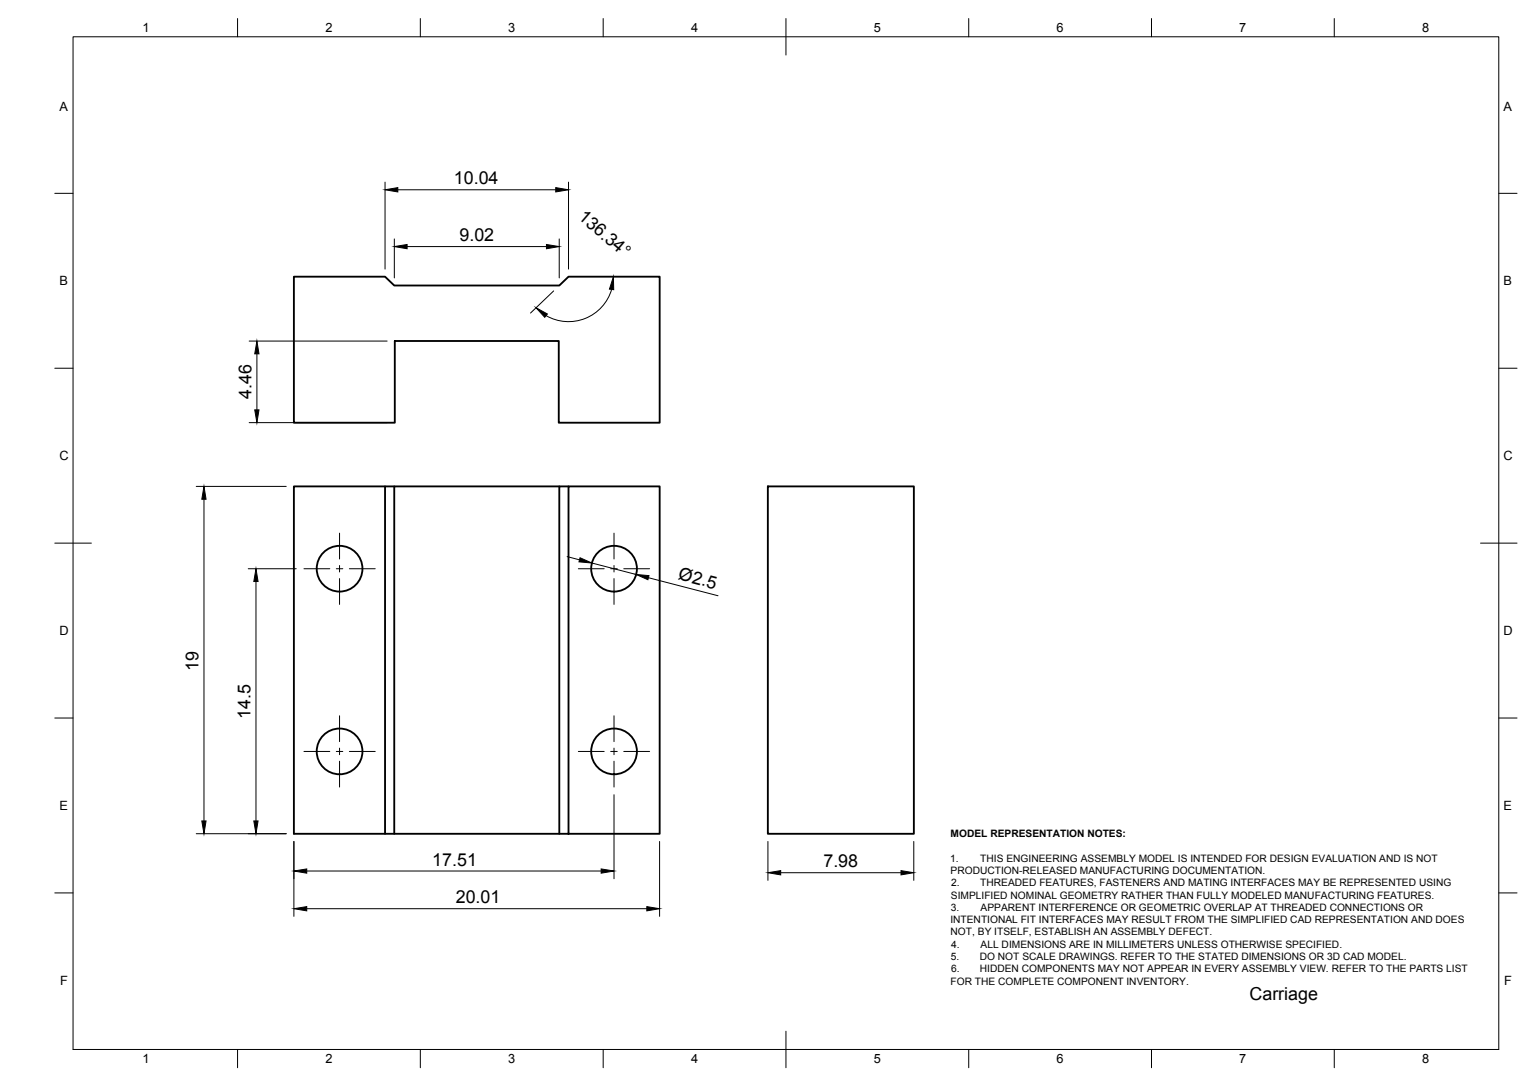
ISO-10303-21;
HEADER;
/* Generated by software containing ST-Developer
 * from STEP Tools, Inc. (www.steptools.com) 
 */

FILE_DESCRIPTION(
/* description */ (''),
/* implementation_level */ '2;1');

FILE_NAME(
/* name */ 'Carriage.step',
/* time_stamp */ '2026-10-06T13:23:02-07:00',
/* author */ (''),
/* organization */ (''),
/* preprocessor_version */ 'ST-DEVELOPER v20.2',
/* originating_system */ 'Autodesk Translation Framework v15.15.0.0',
/* authorisation */ '');

FILE_SCHEMA (('AUTOMOTIVE_DESIGN { 1 0 10303 214 3 1 1 }'));
ENDSEC;

DATA;
#10=MECHANICAL_DESIGN_GEOMETRIC_PRESENTATION_REPRESENTATION('',(#76),#4994);
#56=SHAPE_REPRESENTATION_RELATIONSHIP('SRR','None',#5037,#66);
#66=ADVANCED_BREP_SHAPE_REPRESENTATION('',(#86),#4989);
#76=STYLED_ITEM('',(#5092),#86);
#86=MANIFOLD_SOLID_BREP('Body1',#2916);
#111=CYLINDRICAL_SURFACE('',#3204,1.25);
#112=CYLINDRICAL_SURFACE('',#3208,1.25);
#113=CYLINDRICAL_SURFACE('',#3212,1.25);
#114=CYLINDRICAL_SURFACE('',#3216,1.25);
#146=FACE_BOUND('',#625,.T.);
#147=FACE_BOUND('',#626,.T.);
#148=FACE_BOUND('',#631,.T.);
#149=FACE_BOUND('',#632,.T.);
#241=PLANE('',#3207);
#242=PLANE('',#3211);
#243=PLANE('',#3215);
#244=PLANE('',#3219);
#245=PLANE('',#3220);
#246=PLANE('',#3221);
#247=PLANE('',#3222);
#248=PLANE('',#3223);
#249=PLANE('',#3224);
#250=PLANE('',#3225);
#251=PLANE('',#3226);
#252=PLANE('',#3227);
#253=PLANE('',#3228);
#254=PLANE('',#3229);
#255=PLANE('',#3230);
#256=PLANE('',#3231);
#257=PLANE('',#3232);
#258=PLANE('',#3233);
#411=FACE_OUTER_BOUND('',#612,.T.);
#412=FACE_OUTER_BOUND('',#613,.T.);
#413=FACE_OUTER_BOUND('',#614,.T.);
#414=FACE_OUTER_BOUND('',#615,.T.);
#415=FACE_OUTER_BOUND('',#616,.T.);
#416=FACE_OUTER_BOUND('',#617,.T.);
#417=FACE_OUTER_BOUND('',#618,.T.);
#418=FACE_OUTER_BOUND('',#619,.T.);
#419=FACE_OUTER_BOUND('',#620,.T.);
#420=FACE_OUTER_BOUND('',#621,.T.);
#421=FACE_OUTER_BOUND('',#622,.T.);
#422=FACE_OUTER_BOUND('',#623,.T.);
#423=FACE_OUTER_BOUND('',#624,.T.);
#424=FACE_OUTER_BOUND('',#627,.T.);
#425=FACE_OUTER_BOUND('',#628,.T.);
#426=FACE_OUTER_BOUND('',#629,.T.);
#427=FACE_OUTER_BOUND('',#630,.T.);
#428=FACE_OUTER_BOUND('',#633,.T.);
#429=FACE_OUTER_BOUND('',#634,.T.);
#430=FACE_OUTER_BOUND('',#635,.T.);
#431=FACE_OUTER_BOUND('',#636,.T.);
#432=FACE_OUTER_BOUND('',#637,.T.);
#612=EDGE_LOOP('',(#2388,#2389,#2390,#2391));
#613=EDGE_LOOP('',(#2392));
#614=EDGE_LOOP('',(#2393,#2394,#2395,#2396));
#615=EDGE_LOOP('',(#2397));
#616=EDGE_LOOP('',(#2398,#2399,#2400,#2401));
#617=EDGE_LOOP('',(#2402));
#618=EDGE_LOOP('',(#2403,#2404,#2405,#2406));
#619=EDGE_LOOP('',(#2407));
#620=EDGE_LOOP('',(#2408,#2409,#2410,#2411,#2412,#2413,#2414,#2415,#2416,
#2417,#2418,#2419));
#621=EDGE_LOOP('',(#2420,#2421,#2422,#2423));
#622=EDGE_LOOP('',(#2424,#2425,#2426,#2427));
#623=EDGE_LOOP('',(#2428,#2429,#2430,#2431));
#624=EDGE_LOOP('',(#2432,#2433,#2434,#2435));
#625=EDGE_LOOP('',(#2436));
#626=EDGE_LOOP('',(#2437));
#627=EDGE_LOOP('',(#2438,#2439,#2440,#2441));
#628=EDGE_LOOP('',(#2442,#2443,#2444,#2445));
#629=EDGE_LOOP('',(#2446,#2447,#2448,#2449));
#630=EDGE_LOOP('',(#2450,#2451,#2452,#2453));
#631=EDGE_LOOP('',(#2454));
#632=EDGE_LOOP('',(#2455));
#633=EDGE_LOOP('',(#2456,#2457,#2458,#2459));
#634=EDGE_LOOP('',(#2460,#2461,#2462,#2463));
#635=EDGE_LOOP('',(#2464,#2465,#2466,#2467));
#636=EDGE_LOOP('',(#2468,#2469,#2470,#2471));
#637=EDGE_LOOP('',(#2472,#2473,#2474,#2475,#2476,#2477,#2478,#2479,#2480,
#2481,#2482,#2483));
#851=LINE('',#4611,#1144);
#852=LINE('',#4618,#1145);
#853=LINE('',#4625,#1146);
#854=LINE('',#4632,#1147);
#855=LINE('',#4638,#1148);
#856=LINE('',#4640,#1149);
#857=LINE('',#4642,#1150);
#858=LINE('',#4644,#1151);
#859=LINE('',#4646,#1152);
#860=LINE('',#4648,#1153);
#861=LINE('',#4650,#1154);
#862=LINE('',#4652,#1155);
#863=LINE('',#4654,#1156);
#864=LINE('',#4656,#1157);
#865=LINE('',#4658,#1158);
#866=LINE('',#4659,#1159);
#867=LINE('',#4662,#1160);
#868=LINE('',#4664,#1161);
#869=LINE('',#4665,#1162);
#870=LINE('',#4668,#1163);
#871=LINE('',#4669,#1164);
#872=LINE('',#4672,#1165);
#873=LINE('',#4673,#1166);
#874=LINE('',#4676,#1167);
#875=LINE('',#4677,#1168);
#876=LINE('',#4680,#1169);
#877=LINE('',#4681,#1170);
#878=LINE('',#4684,#1171);
#879=LINE('',#4685,#1172);
#880=LINE('',#4688,#1173);
#881=LINE('',#4689,#1174);
#882=LINE('',#4692,#1175);
#883=LINE('',#4693,#1176);
#884=LINE('',#4696,#1177);
#885=LINE('',#4697,#1178);
#886=LINE('',#4700,#1179);
#887=LINE('',#4701,#1180);
#888=LINE('',#4704,#1181);
#889=LINE('',#4705,#1182);
#890=LINE('',#4707,#1183);
#1144=VECTOR('',#3809,1.25);
#1145=VECTOR('',#3818,1.25);
#1146=VECTOR('',#3827,1.25);
#1147=VECTOR('',#3836,1.25);
#1148=VECTOR('',#3843,10.);
#1149=VECTOR('',#3844,10.);
#1150=VECTOR('',#3845,10.);
#1151=VECTOR('',#3846,10.);
#1152=VECTOR('',#3847,10.);
#1153=VECTOR('',#3848,10.);
#1154=VECTOR('',#3849,10.);
#1155=VECTOR('',#3850,10.);
#1156=VECTOR('',#3851,10.);
#1157=VECTOR('',#3852,10.);
#1158=VECTOR('',#3853,10.);
#1159=VECTOR('',#3854,10.);
#1160=VECTOR('',#3857,10.);
#1161=VECTOR('',#3858,10.);
#1162=VECTOR('',#3859,10.);
#1163=VECTOR('',#3862,10.);
#1164=VECTOR('',#3863,10.);
#1165=VECTOR('',#3866,10.);
#1166=VECTOR('',#3867,10.);
#1167=VECTOR('',#3870,10.);
#1168=VECTOR('',#3871,10.);
#1169=VECTOR('',#3874,10.);
#1170=VECTOR('',#3875,10.);
#1171=VECTOR('',#3878,10.);
#1172=VECTOR('',#3879,10.);
#1173=VECTOR('',#3882,10.);
#1174=VECTOR('',#3883,10.);
#1175=VECTOR('',#3886,10.);
#1176=VECTOR('',#3887,10.);
#1177=VECTOR('',#3890,10.);
#1178=VECTOR('',#3891,10.);
#1179=VECTOR('',#3894,10.);
#1180=VECTOR('',#3895,10.);
#1181=VECTOR('',#3898,10.);
#1182=VECTOR('',#3899,10.);
#1183=VECTOR('',#3902,10.);
#1345=CIRCLE('',#3205,1.25);
#1346=CIRCLE('',#3206,1.25);
#1347=CIRCLE('',#3209,1.25);
#1348=CIRCLE('',#3210,1.25);
#1349=CIRCLE('',#3213,1.25);
#1350=CIRCLE('',#3214,1.25);
#1351=CIRCLE('',#3217,1.25);
#1352=CIRCLE('',#3218,1.25);
#1490=VERTEX_POINT('',#4608);
#1491=VERTEX_POINT('',#4610);
#1492=VERTEX_POINT('',#4615);
#1493=VERTEX_POINT('',#4617);
#1494=VERTEX_POINT('',#4622);
#1495=VERTEX_POINT('',#4624);
#1496=VERTEX_POINT('',#4629);
#1497=VERTEX_POINT('',#4631);
#1498=VERTEX_POINT('',#4636);
#1499=VERTEX_POINT('',#4637);
#1500=VERTEX_POINT('',#4639);
#1501=VERTEX_POINT('',#4641);
#1502=VERTEX_POINT('',#4643);
#1503=VERTEX_POINT('',#4645);
#1504=VERTEX_POINT('',#4647);
#1505=VERTEX_POINT('',#4649);
#1506=VERTEX_POINT('',#4651);
#1507=VERTEX_POINT('',#4653);
#1508=VERTEX_POINT('',#4655);
#1509=VERTEX_POINT('',#4657);
#1510=VERTEX_POINT('',#4661);
#1511=VERTEX_POINT('',#4663);
#1512=VERTEX_POINT('',#4667);
#1513=VERTEX_POINT('',#4671);
#1514=VERTEX_POINT('',#4675);
#1515=VERTEX_POINT('',#4679);
#1516=VERTEX_POINT('',#4683);
#1517=VERTEX_POINT('',#4687);
#1518=VERTEX_POINT('',#4691);
#1519=VERTEX_POINT('',#4695);
#1520=VERTEX_POINT('',#4699);
#1521=VERTEX_POINT('',#4703);
#1808=EDGE_CURVE('',#1490,#1490,#1345,.T.);
#1809=EDGE_CURVE('',#1490,#1491,#851,.T.);
#1810=EDGE_CURVE('',#1491,#1491,#1346,.T.);
#1811=EDGE_CURVE('',#1492,#1492,#1347,.T.);
#1812=EDGE_CURVE('',#1492,#1493,#852,.T.);
#1813=EDGE_CURVE('',#1493,#1493,#1348,.T.);
#1814=EDGE_CURVE('',#1494,#1494,#1349,.T.);
#1815=EDGE_CURVE('',#1494,#1495,#853,.T.);
#1816=EDGE_CURVE('',#1495,#1495,#1350,.T.);
#1817=EDGE_CURVE('',#1496,#1496,#1351,.T.);
#1818=EDGE_CURVE('',#1496,#1497,#854,.T.);
#1819=EDGE_CURVE('',#1497,#1497,#1352,.T.);
#1820=EDGE_CURVE('',#1498,#1499,#855,.T.);
#1821=EDGE_CURVE('',#1499,#1500,#856,.T.);
#1822=EDGE_CURVE('',#1500,#1501,#857,.T.);
#1823=EDGE_CURVE('',#1501,#1502,#858,.T.);
#1824=EDGE_CURVE('',#1502,#1503,#859,.T.);
#1825=EDGE_CURVE('',#1503,#1504,#860,.T.);
#1826=EDGE_CURVE('',#1504,#1505,#861,.T.);
#1827=EDGE_CURVE('',#1505,#1506,#862,.T.);
#1828=EDGE_CURVE('',#1506,#1507,#863,.T.);
#1829=EDGE_CURVE('',#1507,#1508,#864,.T.);
#1830=EDGE_CURVE('',#1508,#1509,#865,.T.);
#1831=EDGE_CURVE('',#1509,#1498,#866,.T.);
#1832=EDGE_CURVE('',#1499,#1510,#867,.T.);
#1833=EDGE_CURVE('',#1511,#1510,#868,.T.);
#1834=EDGE_CURVE('',#1500,#1511,#869,.T.);
#1835=EDGE_CURVE('',#1512,#1511,#870,.T.);
#1836=EDGE_CURVE('',#1501,#1512,#871,.T.);
#1837=EDGE_CURVE('',#1513,#1512,#872,.T.);
#1838=EDGE_CURVE('',#1502,#1513,#873,.T.);
#1839=EDGE_CURVE('',#1514,#1513,#874,.T.);
#1840=EDGE_CURVE('',#1503,#1514,#875,.T.);
#1841=EDGE_CURVE('',#1515,#1514,#876,.T.);
#1842=EDGE_CURVE('',#1504,#1515,#877,.T.);
#1843=EDGE_CURVE('',#1516,#1515,#878,.T.);
#1844=EDGE_CURVE('',#1505,#1516,#879,.T.);
#1845=EDGE_CURVE('',#1517,#1516,#880,.T.);
#1846=EDGE_CURVE('',#1506,#1517,#881,.T.);
#1847=EDGE_CURVE('',#1518,#1517,#882,.T.);
#1848=EDGE_CURVE('',#1507,#1518,#883,.T.);
#1849=EDGE_CURVE('',#1519,#1518,#884,.T.);
#1850=EDGE_CURVE('',#1508,#1519,#885,.T.);
#1851=EDGE_CURVE('',#1520,#1519,#886,.T.);
#1852=EDGE_CURVE('',#1509,#1520,#887,.T.);
#1853=EDGE_CURVE('',#1521,#1520,#888,.T.);
#1854=EDGE_CURVE('',#1498,#1521,#889,.T.);
#1855=EDGE_CURVE('',#1510,#1521,#890,.T.);
#2388=ORIENTED_EDGE('',*,*,#1808,.F.);
#2389=ORIENTED_EDGE('',*,*,#1809,.T.);
#2390=ORIENTED_EDGE('',*,*,#1810,.T.);
#2391=ORIENTED_EDGE('',*,*,#1809,.F.);
#2392=ORIENTED_EDGE('',*,*,#1810,.F.);
#2393=ORIENTED_EDGE('',*,*,#1811,.F.);
#2394=ORIENTED_EDGE('',*,*,#1812,.T.);
#2395=ORIENTED_EDGE('',*,*,#1813,.T.);
#2396=ORIENTED_EDGE('',*,*,#1812,.F.);
#2397=ORIENTED_EDGE('',*,*,#1813,.F.);
#2398=ORIENTED_EDGE('',*,*,#1814,.F.);
#2399=ORIENTED_EDGE('',*,*,#1815,.T.);
#2400=ORIENTED_EDGE('',*,*,#1816,.T.);
#2401=ORIENTED_EDGE('',*,*,#1815,.F.);
#2402=ORIENTED_EDGE('',*,*,#1816,.F.);
#2403=ORIENTED_EDGE('',*,*,#1817,.F.);
#2404=ORIENTED_EDGE('',*,*,#1818,.T.);
#2405=ORIENTED_EDGE('',*,*,#1819,.T.);
#2406=ORIENTED_EDGE('',*,*,#1818,.F.);
#2407=ORIENTED_EDGE('',*,*,#1819,.F.);
#2408=ORIENTED_EDGE('',*,*,#1820,.T.);
#2409=ORIENTED_EDGE('',*,*,#1821,.T.);
#2410=ORIENTED_EDGE('',*,*,#1822,.T.);
#2411=ORIENTED_EDGE('',*,*,#1823,.T.);
#2412=ORIENTED_EDGE('',*,*,#1824,.T.);
#2413=ORIENTED_EDGE('',*,*,#1825,.T.);
#2414=ORIENTED_EDGE('',*,*,#1826,.T.);
#2415=ORIENTED_EDGE('',*,*,#1827,.T.);
#2416=ORIENTED_EDGE('',*,*,#1828,.T.);
#2417=ORIENTED_EDGE('',*,*,#1829,.T.);
#2418=ORIENTED_EDGE('',*,*,#1830,.T.);
#2419=ORIENTED_EDGE('',*,*,#1831,.T.);
#2420=ORIENTED_EDGE('',*,*,#1832,.T.);
#2421=ORIENTED_EDGE('',*,*,#1833,.F.);
#2422=ORIENTED_EDGE('',*,*,#1834,.F.);
#2423=ORIENTED_EDGE('',*,*,#1821,.F.);
#2424=ORIENTED_EDGE('',*,*,#1834,.T.);
#2425=ORIENTED_EDGE('',*,*,#1835,.F.);
#2426=ORIENTED_EDGE('',*,*,#1836,.F.);
#2427=ORIENTED_EDGE('',*,*,#1822,.F.);
#2428=ORIENTED_EDGE('',*,*,#1836,.T.);
#2429=ORIENTED_EDGE('',*,*,#1837,.F.);
#2430=ORIENTED_EDGE('',*,*,#1838,.F.);
#2431=ORIENTED_EDGE('',*,*,#1823,.F.);
#2432=ORIENTED_EDGE('',*,*,#1838,.T.);
#2433=ORIENTED_EDGE('',*,*,#1839,.F.);
#2434=ORIENTED_EDGE('',*,*,#1840,.F.);
#2435=ORIENTED_EDGE('',*,*,#1824,.F.);
#2436=ORIENTED_EDGE('',*,*,#1808,.T.);
#2437=ORIENTED_EDGE('',*,*,#1814,.T.);
#2438=ORIENTED_EDGE('',*,*,#1840,.T.);
#2439=ORIENTED_EDGE('',*,*,#1841,.F.);
#2440=ORIENTED_EDGE('',*,*,#1842,.F.);
#2441=ORIENTED_EDGE('',*,*,#1825,.F.);
#2442=ORIENTED_EDGE('',*,*,#1842,.T.);
#2443=ORIENTED_EDGE('',*,*,#1843,.F.);
#2444=ORIENTED_EDGE('',*,*,#1844,.F.);
#2445=ORIENTED_EDGE('',*,*,#1826,.F.);
#2446=ORIENTED_EDGE('',*,*,#1844,.T.);
#2447=ORIENTED_EDGE('',*,*,#1845,.F.);
#2448=ORIENTED_EDGE('',*,*,#1846,.F.);
#2449=ORIENTED_EDGE('',*,*,#1827,.F.);
#2450=ORIENTED_EDGE('',*,*,#1846,.T.);
#2451=ORIENTED_EDGE('',*,*,#1847,.F.);
#2452=ORIENTED_EDGE('',*,*,#1848,.F.);
#2453=ORIENTED_EDGE('',*,*,#1828,.F.);
#2454=ORIENTED_EDGE('',*,*,#1811,.T.);
#2455=ORIENTED_EDGE('',*,*,#1817,.T.);
#2456=ORIENTED_EDGE('',*,*,#1848,.T.);
#2457=ORIENTED_EDGE('',*,*,#1849,.F.);
#2458=ORIENTED_EDGE('',*,*,#1850,.F.);
#2459=ORIENTED_EDGE('',*,*,#1829,.F.);
#2460=ORIENTED_EDGE('',*,*,#1850,.T.);
#2461=ORIENTED_EDGE('',*,*,#1851,.F.);
#2462=ORIENTED_EDGE('',*,*,#1852,.F.);
#2463=ORIENTED_EDGE('',*,*,#1830,.F.);
#2464=ORIENTED_EDGE('',*,*,#1852,.T.);
#2465=ORIENTED_EDGE('',*,*,#1853,.F.);
#2466=ORIENTED_EDGE('',*,*,#1854,.F.);
#2467=ORIENTED_EDGE('',*,*,#1831,.F.);
#2468=ORIENTED_EDGE('',*,*,#1854,.T.);
#2469=ORIENTED_EDGE('',*,*,#1855,.F.);
#2470=ORIENTED_EDGE('',*,*,#1832,.F.);
#2471=ORIENTED_EDGE('',*,*,#1820,.F.);
#2472=ORIENTED_EDGE('',*,*,#1855,.T.);
#2473=ORIENTED_EDGE('',*,*,#1853,.T.);
#2474=ORIENTED_EDGE('',*,*,#1851,.T.);
#2475=ORIENTED_EDGE('',*,*,#1849,.T.);
#2476=ORIENTED_EDGE('',*,*,#1847,.T.);
#2477=ORIENTED_EDGE('',*,*,#1845,.T.);
#2478=ORIENTED_EDGE('',*,*,#1843,.T.);
#2479=ORIENTED_EDGE('',*,*,#1841,.T.);
#2480=ORIENTED_EDGE('',*,*,#1839,.T.);
#2481=ORIENTED_EDGE('',*,*,#1837,.T.);
#2482=ORIENTED_EDGE('',*,*,#1835,.T.);
#2483=ORIENTED_EDGE('',*,*,#1833,.T.);
#2841=ADVANCED_FACE('',(#411),#111,.F.);
#2842=ADVANCED_FACE('',(#412),#241,.T.);
#2843=ADVANCED_FACE('',(#413),#112,.F.);
#2844=ADVANCED_FACE('',(#414),#242,.T.);
#2845=ADVANCED_FACE('',(#415),#113,.F.);
#2846=ADVANCED_FACE('',(#416),#243,.T.);
#2847=ADVANCED_FACE('',(#417),#114,.F.);
#2848=ADVANCED_FACE('',(#418),#244,.T.);
#2849=ADVANCED_FACE('',(#419),#245,.T.);
#2850=ADVANCED_FACE('',(#420),#246,.T.);
#2851=ADVANCED_FACE('',(#421),#247,.T.);
#2852=ADVANCED_FACE('',(#422),#248,.T.);
#2853=ADVANCED_FACE('',(#423,#146,#147),#249,.T.);
#2854=ADVANCED_FACE('',(#424),#250,.T.);
#2855=ADVANCED_FACE('',(#425),#251,.T.);
#2856=ADVANCED_FACE('',(#426),#252,.T.);
#2857=ADVANCED_FACE('',(#427,#148,#149),#253,.T.);
#2858=ADVANCED_FACE('',(#428),#254,.T.);
#2859=ADVANCED_FACE('',(#429),#255,.T.);
#2860=ADVANCED_FACE('',(#430),#256,.T.);
#2861=ADVANCED_FACE('',(#431),#257,.T.);
#2862=ADVANCED_FACE('',(#432),#258,.T.);
#2916=CLOSED_SHELL('',(#2841,#2842,#2843,#2844,#2845,#2846,#2847,#2848,
#2849,#2850,#2851,#2852,#2853,#2854,#2855,#2856,#2857,#2858,#2859,#2860,
#2861,#2862));
#3203=AXIS2_PLACEMENT_3D('',#4606,#3803,#3804);
#3204=AXIS2_PLACEMENT_3D('',#4607,#3805,#3806);
#3205=AXIS2_PLACEMENT_3D('',#4609,#3807,#3808);
#3206=AXIS2_PLACEMENT_3D('',#4612,#3810,#3811);
#3207=AXIS2_PLACEMENT_3D('',#4613,#3812,#3813);
#3208=AXIS2_PLACEMENT_3D('',#4614,#3814,#3815);
#3209=AXIS2_PLACEMENT_3D('',#4616,#3816,#3817);
#3210=AXIS2_PLACEMENT_3D('',#4619,#3819,#3820);
#3211=AXIS2_PLACEMENT_3D('',#4620,#3821,#3822);
#3212=AXIS2_PLACEMENT_3D('',#4621,#3823,#3824);
#3213=AXIS2_PLACEMENT_3D('',#4623,#3825,#3826);
#3214=AXIS2_PLACEMENT_3D('',#4626,#3828,#3829);
#3215=AXIS2_PLACEMENT_3D('',#4627,#3830,#3831);
#3216=AXIS2_PLACEMENT_3D('',#4628,#3832,#3833);
#3217=AXIS2_PLACEMENT_3D('',#4630,#3834,#3835);
#3218=AXIS2_PLACEMENT_3D('',#4633,#3837,#3838);
#3219=AXIS2_PLACEMENT_3D('',#4634,#3839,#3840);
#3220=AXIS2_PLACEMENT_3D('',#4635,#3841,#3842);
#3221=AXIS2_PLACEMENT_3D('',#4660,#3855,#3856);
#3222=AXIS2_PLACEMENT_3D('',#4666,#3860,#3861);
#3223=AXIS2_PLACEMENT_3D('',#4670,#3864,#3865);
#3224=AXIS2_PLACEMENT_3D('',#4674,#3868,#3869);
#3225=AXIS2_PLACEMENT_3D('',#4678,#3872,#3873);
#3226=AXIS2_PLACEMENT_3D('',#4682,#3876,#3877);
#3227=AXIS2_PLACEMENT_3D('',#4686,#3880,#3881);
#3228=AXIS2_PLACEMENT_3D('',#4690,#3884,#3885);
#3229=AXIS2_PLACEMENT_3D('',#4694,#3888,#3889);
#3230=AXIS2_PLACEMENT_3D('',#4698,#3892,#3893);
#3231=AXIS2_PLACEMENT_3D('',#4702,#3896,#3897);
#3232=AXIS2_PLACEMENT_3D('',#4706,#3900,#3901);
#3233=AXIS2_PLACEMENT_3D('',#4708,#3903,#3904);
#3803=DIRECTION('axis',(0.,0.,1.));
#3804=DIRECTION('refdir',(1.,0.,0.));
#3805=DIRECTION('center_axis',(0.,0.,-1.));
#3806=DIRECTION('ref_axis',(-1.,0.,0.));
#3807=DIRECTION('center_axis',(0.,0.,-1.));
#3808=DIRECTION('ref_axis',(-1.,0.,0.));
#3809=DIRECTION('',(0.,0.,-1.));
#3810=DIRECTION('center_axis',(0.,0.,-1.));
#3811=DIRECTION('ref_axis',(-1.,0.,0.));
#3812=DIRECTION('center_axis',(0.,0.,1.));
#3813=DIRECTION('ref_axis',(-1.,0.,0.));
#3814=DIRECTION('center_axis',(0.,0.,-1.));
#3815=DIRECTION('ref_axis',(-1.,0.,0.));
#3816=DIRECTION('center_axis',(0.,0.,-1.));
#3817=DIRECTION('ref_axis',(-1.,0.,0.));
#3818=DIRECTION('',(0.,0.,-1.));
#3819=DIRECTION('center_axis',(0.,0.,-1.));
#3820=DIRECTION('ref_axis',(-1.,0.,0.));
#3821=DIRECTION('center_axis',(0.,0.,1.));
#3822=DIRECTION('ref_axis',(-1.,0.,0.));
#3823=DIRECTION('center_axis',(0.,0.,-1.));
#3824=DIRECTION('ref_axis',(-1.,0.,0.));
#3825=DIRECTION('center_axis',(0.,0.,-1.));
#3826=DIRECTION('ref_axis',(-1.,0.,0.));
#3827=DIRECTION('',(0.,0.,-1.));
#3828=DIRECTION('center_axis',(0.,0.,-1.));
#3829=DIRECTION('ref_axis',(-1.,0.,0.));
#3830=DIRECTION('center_axis',(0.,0.,1.));
#3831=DIRECTION('ref_axis',(-1.,0.,0.));
#3832=DIRECTION('center_axis',(0.,0.,-1.));
#3833=DIRECTION('ref_axis',(-1.,0.,0.));
#3834=DIRECTION('center_axis',(0.,0.,-1.));
#3835=DIRECTION('ref_axis',(-1.,0.,0.));
#3836=DIRECTION('',(0.,0.,-1.));
#3837=DIRECTION('center_axis',(0.,0.,-1.));
#3838=DIRECTION('ref_axis',(-1.,0.,0.));
#3839=DIRECTION('center_axis',(0.,0.,1.));
#3840=DIRECTION('ref_axis',(-1.,0.,0.));
#3841=DIRECTION('center_axis',(-1.,0.,0.));
#3842=DIRECTION('ref_axis',(0.,0.,1.));
#3843=DIRECTION('',(0.,-1.,0.));
#3844=DIRECTION('',(0.,0.,-1.));
#3845=DIRECTION('',(0.,-1.,0.));
#3846=DIRECTION('',(0.,0.,1.));
#3847=DIRECTION('',(0.,1.,0.));
#3848=DIRECTION('',(0.,0.723499719481454,-0.690324674273097));
#3849=DIRECTION('',(0.,1.,0.));
#3850=DIRECTION('',(0.,0.723499719481453,0.690324674273098));
#3851=DIRECTION('',(0.,1.,0.));
#3852=DIRECTION('',(0.,0.,-1.));
#3853=DIRECTION('',(0.,-1.,0.));
#3854=DIRECTION('',(0.,0.,1.));
#3855=DIRECTION('center_axis',(0.,1.,0.));
#3856=DIRECTION('ref_axis',(0.,0.,1.));
#3857=DIRECTION('',(1.,0.,0.));
#3858=DIRECTION('',(0.,0.,1.));
#3859=DIRECTION('',(1.,0.,0.));
#3860=DIRECTION('center_axis',(0.,0.,-1.));
#3861=DIRECTION('ref_axis',(0.,1.,0.));
#3862=DIRECTION('',(0.,1.,0.));
#3863=DIRECTION('',(1.,0.,0.));
#3864=DIRECTION('center_axis',(0.,-1.,0.));
#3865=DIRECTION('ref_axis',(0.,0.,-1.));
#3866=DIRECTION('',(0.,0.,-1.));
#3867=DIRECTION('',(1.,0.,0.));
#3868=DIRECTION('center_axis',(0.,0.,1.));
#3869=DIRECTION('ref_axis',(0.,-1.,0.));
#3870=DIRECTION('',(0.,-1.,0.));
#3871=DIRECTION('',(1.,0.,0.));
#3872=DIRECTION('center_axis',(0.,0.690324674273097,0.723499719481454));
#3873=DIRECTION('ref_axis',(0.,-0.723499719481454,0.690324674273097));
#3874=DIRECTION('',(0.,-0.723499719481454,0.690324674273097));
#3875=DIRECTION('',(1.,0.,0.));
#3876=DIRECTION('center_axis',(0.,0.,1.));
#3877=DIRECTION('ref_axis',(0.,-1.,0.));
#3878=DIRECTION('',(0.,-1.,0.));
#3879=DIRECTION('',(1.,0.,0.));
#3880=DIRECTION('center_axis',(0.,-0.690324674273098,0.723499719481453));
#3881=DIRECTION('ref_axis',(0.,-0.723499719481453,-0.690324674273098));
#3882=DIRECTION('',(0.,-0.723499719481453,-0.690324674273098));
#3883=DIRECTION('',(1.,0.,0.));
#3884=DIRECTION('center_axis',(0.,0.,1.));
#3885=DIRECTION('ref_axis',(0.,-1.,0.));
#3886=DIRECTION('',(0.,-1.,0.));
#3887=DIRECTION('',(1.,0.,0.));
#3888=DIRECTION('center_axis',(0.,1.,0.));
#3889=DIRECTION('ref_axis',(0.,0.,1.));
#3890=DIRECTION('',(0.,0.,1.));
#3891=DIRECTION('',(1.,0.,0.));
#3892=DIRECTION('center_axis',(0.,0.,-1.));
#3893=DIRECTION('ref_axis',(0.,1.,0.));
#3894=DIRECTION('',(0.,1.,0.));
#3895=DIRECTION('',(1.,0.,0.));
#3896=DIRECTION('center_axis',(0.,-1.,0.));
#3897=DIRECTION('ref_axis',(0.,0.,-1.));
#3898=DIRECTION('',(0.,0.,-1.));
#3899=DIRECTION('',(1.,0.,0.));
#3900=DIRECTION('center_axis',(0.,0.,-1.));
#3901=DIRECTION('ref_axis',(0.,1.,0.));
#3902=DIRECTION('',(0.,1.,0.));
#3903=DIRECTION('center_axis',(1.,0.,0.));
#3904=DIRECTION('ref_axis',(0.,0.,-1.));
#4606=CARTESIAN_POINT('',(0.,0.,0.));
#4607=CARTESIAN_POINT('Origin',(4.99661841059868,-7.50651000176462,6.74711402388884));
#4608=CARTESIAN_POINT('',(6.24661841059868,-7.50651000176462,6.74711402388884));
#4609=CARTESIAN_POINT('Origin',(4.99661841059868,-7.50651000176462,6.74711402388884));
#4610=CARTESIAN_POINT('',(6.24661841059868,-7.50651000176462,1.74711402388884));
#4611=CARTESIAN_POINT('',(6.24661841059868,-7.50651000176462,6.74711402388884));
#4612=CARTESIAN_POINT('Origin',(4.99661841059868,-7.50651000176462,1.74711402388884));
#4613=CARTESIAN_POINT('Origin',(4.99661841059868,-7.50651000176462,1.74711402388884));
#4614=CARTESIAN_POINT('Origin',(-4.99661841059868,7.50651000176462,6.74711402388884));
#4615=CARTESIAN_POINT('',(-3.74661841059868,7.50651000176462,6.74711402388884));
#4616=CARTESIAN_POINT('Origin',(-4.99661841059868,7.50651000176462,6.74711402388884));
#4617=CARTESIAN_POINT('',(-3.74661841059868,7.50651000176462,1.74711402388884));
#4618=CARTESIAN_POINT('',(-3.74661841059868,7.50651000176462,6.74711402388884));
#4619=CARTESIAN_POINT('Origin',(-4.99661841059868,7.50651000176462,1.74711402388884));
#4620=CARTESIAN_POINT('Origin',(-4.99661841059868,7.50651000176462,1.74711402388884));
#4621=CARTESIAN_POINT('Origin',(-4.99661841059868,-7.50651000176462,6.74711402388884));
#4622=CARTESIAN_POINT('',(-3.74661841059868,-7.50651000176462,6.74711402388884));
#4623=CARTESIAN_POINT('Origin',(-4.99661841059868,-7.50651000176462,6.74711402388884));
#4624=CARTESIAN_POINT('',(-3.74661841059868,-7.50651000176462,1.74711402388884));
#4625=CARTESIAN_POINT('',(-3.74661841059868,-7.50651000176462,6.74711402388884));
#4626=CARTESIAN_POINT('Origin',(-4.99661841059868,-7.50651000176462,1.74711402388884));
#4627=CARTESIAN_POINT('Origin',(-4.99661841059868,-7.50651000176462,1.74711402388884));
#4628=CARTESIAN_POINT('Origin',(4.99661841059868,7.50651000176462,6.74711402388884));
#4629=CARTESIAN_POINT('',(6.24661841059868,7.50651000176462,6.74711402388884));
#4630=CARTESIAN_POINT('Origin',(4.99661841059868,7.50651000176462,6.74711402388884));
#4631=CARTESIAN_POINT('',(6.24661841059868,7.50651000176462,1.74711402388884));
#4632=CARTESIAN_POINT('',(6.24661841059868,7.50651000176462,6.74711402388884));
#4633=CARTESIAN_POINT('Origin',(4.99661841059868,7.50651000176462,1.74711402388884));
#4634=CARTESIAN_POINT('Origin',(4.99661841059868,7.50651000176462,1.74711402388884));
#4635=CARTESIAN_POINT('Origin',(-9.5,0.,2.75621475582567));
#4636=CARTESIAN_POINT('',(-9.5,4.48396394323217,3.23022961141938));
#4637=CARTESIAN_POINT('',(-9.5,-4.48396394323217,3.23022961141938));
#4638=CARTESIAN_POINT('',(-9.5,0.,3.23022961141938));
#4639=CARTESIAN_POINT('',(-9.5,-4.48396394323217,-1.2346845122375));
#4640=CARTESIAN_POINT('',(-9.5,-4.48396394323217,3.23022961141938));
#4641=CARTESIAN_POINT('',(-9.5,-10.0039433906299,-1.2346845122375));
#4642=CARTESIAN_POINT('',(-9.5,-4.48396394323217,-1.2346845122375));
#4643=CARTESIAN_POINT('',(-9.5,-10.0039433906299,6.74711402388884));
#4644=CARTESIAN_POINT('',(-9.5,-10.0039433906299,-1.2346845122375));
#4645=CARTESIAN_POINT('',(-9.5,-5.01914200599926,6.74711402388884));
#4646=CARTESIAN_POINT('',(-9.5,-10.0039433906299,6.74711402388884));
#4647=CARTESIAN_POINT('',(-9.5,-4.51226721735165,6.26348125396712));
#4648=CARTESIAN_POINT('',(-9.5,-5.01914200599926,6.74711402388884));
#4649=CARTESIAN_POINT('',(-9.5,4.51226721735165,6.26348125396712));
#4650=CARTESIAN_POINT('',(-9.5,4.51226721735165,6.26348125396712));
#4651=CARTESIAN_POINT('',(-9.5,5.01914200599926,6.74711402388884));
#4652=CARTESIAN_POINT('',(-9.5,5.01914200599926,6.74711402388884));
#4653=CARTESIAN_POINT('',(-9.5,10.0039433906299,6.74711402388884));
#4654=CARTESIAN_POINT('',(-9.5,10.0039433906299,6.74711402388884));
#4655=CARTESIAN_POINT('',(-9.5,10.0039433906299,-1.2346845122375));
#4656=CARTESIAN_POINT('',(-9.5,10.0039433906299,-1.2346845122375));
#4657=CARTESIAN_POINT('',(-9.5,4.48396394323217,-1.2346845122375));
#4658=CARTESIAN_POINT('',(-9.5,4.48396394323217,-1.2346845122375));
#4659=CARTESIAN_POINT('',(-9.5,4.48396394323217,3.23022961141938));
#4660=CARTESIAN_POINT('Origin',(0.,-4.48396394323217,-1.2346845122375));
#4661=CARTESIAN_POINT('',(9.5,-4.48396394323217,3.23022961141938));
#4662=CARTESIAN_POINT('',(0.,-4.48396394323217,3.23022961141938));
#4663=CARTESIAN_POINT('',(9.5,-4.48396394323217,-1.2346845122375));
#4664=CARTESIAN_POINT('',(9.5,-4.48396394323217,3.23022961141938));
#4665=CARTESIAN_POINT('',(0.,-4.48396394323217,-1.2346845122375));
#4666=CARTESIAN_POINT('Origin',(0.,-10.0039433906299,-1.2346845122375));
#4667=CARTESIAN_POINT('',(9.5,-10.0039433906299,-1.2346845122375));
#4668=CARTESIAN_POINT('',(9.5,-4.48396394323217,-1.2346845122375));
#4669=CARTESIAN_POINT('',(0.,-10.0039433906299,-1.2346845122375));
#4670=CARTESIAN_POINT('Origin',(0.,-10.0039433906299,6.74711402388884));
#4671=CARTESIAN_POINT('',(9.5,-10.0039433906299,6.74711402388884));
#4672=CARTESIAN_POINT('',(9.5,-10.0039433906299,-1.2346845122375));
#4673=CARTESIAN_POINT('',(0.,-10.0039433906299,6.74711402388884));
#4674=CARTESIAN_POINT('Origin',(0.,-5.01914200599926,6.74711402388884));
#4675=CARTESIAN_POINT('',(9.5,-5.01914200599926,6.74711402388884));
#4676=CARTESIAN_POINT('',(9.5,-10.0039433906299,6.74711402388884));
#4677=CARTESIAN_POINT('',(0.,-5.01914200599926,6.74711402388884));
#4678=CARTESIAN_POINT('Origin',(0.,-4.51226721735165,6.26348125396712));
#4679=CARTESIAN_POINT('',(9.5,-4.51226721735165,6.26348125396712));
#4680=CARTESIAN_POINT('',(9.5,-5.01914200599926,6.74711402388884));
#4681=CARTESIAN_POINT('',(0.,-4.51226721735165,6.26348125396712));
#4682=CARTESIAN_POINT('Origin',(0.,4.51226721735165,6.26348125396712));
#4683=CARTESIAN_POINT('',(9.5,4.51226721735165,6.26348125396712));
#4684=CARTESIAN_POINT('',(9.5,4.51226721735165,6.26348125396712));
#4685=CARTESIAN_POINT('',(0.,4.51226721735165,6.26348125396712));
#4686=CARTESIAN_POINT('Origin',(0.,5.01914200599926,6.74711402388884));
#4687=CARTESIAN_POINT('',(9.5,5.01914200599926,6.74711402388884));
#4688=CARTESIAN_POINT('',(9.5,5.01914200599926,6.74711402388884));
#4689=CARTESIAN_POINT('',(0.,5.01914200599926,6.74711402388884));
#4690=CARTESIAN_POINT('Origin',(0.,10.0039433906299,6.74711402388884));
#4691=CARTESIAN_POINT('',(9.5,10.0039433906299,6.74711402388884));
#4692=CARTESIAN_POINT('',(9.5,10.0039433906299,6.74711402388884));
#4693=CARTESIAN_POINT('',(0.,10.0039433906299,6.74711402388884));
#4694=CARTESIAN_POINT('Origin',(0.,10.0039433906299,-1.2346845122375));
#4695=CARTESIAN_POINT('',(9.5,10.0039433906299,-1.2346845122375));
#4696=CARTESIAN_POINT('',(9.5,10.0039433906299,-1.2346845122375));
#4697=CARTESIAN_POINT('',(0.,10.0039433906299,-1.2346845122375));
#4698=CARTESIAN_POINT('Origin',(0.,4.48396394323217,-1.2346845122375));
#4699=CARTESIAN_POINT('',(9.5,4.48396394323217,-1.2346845122375));
#4700=CARTESIAN_POINT('',(9.5,4.48396394323217,-1.2346845122375));
#4701=CARTESIAN_POINT('',(0.,4.48396394323217,-1.2346845122375));
#4702=CARTESIAN_POINT('Origin',(0.,4.48396394323217,3.23022961141938));
#4703=CARTESIAN_POINT('',(9.5,4.48396394323217,3.23022961141938));
#4704=CARTESIAN_POINT('',(9.5,4.48396394323217,3.23022961141938));
#4705=CARTESIAN_POINT('',(0.,4.48396394323217,3.23022961141938));
#4706=CARTESIAN_POINT('Origin',(0.,-4.48396394323217,3.23022961141938));
#4707=CARTESIAN_POINT('',(9.5,0.,3.23022961141938));
#4708=CARTESIAN_POINT('Origin',(9.5,0.,2.75621475582567));
#4977=UNCERTAINTY_MEASURE_WITH_UNIT(LENGTH_MEASURE(0.01),#4995,
'DISTANCE_ACCURACY_VALUE',
'Maximum model space distance between geometric entities at asserted c
onnectivities');
#4982=UNCERTAINTY_MEASURE_WITH_UNIT(LENGTH_MEASURE(0.01),#4995,
'DISTANCE_ACCURACY_VALUE',
'Maximum model space distance between geometric entities at asserted c
onnectivities');
#4989=(
GEOMETRIC_REPRESENTATION_CONTEXT(3)
GLOBAL_UNCERTAINTY_ASSIGNED_CONTEXT((#4977))
GLOBAL_UNIT_ASSIGNED_CONTEXT((#4995,#4997,#4998))
REPRESENTATION_CONTEXT('','3D')
);
#4994=(
GEOMETRIC_REPRESENTATION_CONTEXT(3)
GLOBAL_UNCERTAINTY_ASSIGNED_CONTEXT((#4982))
GLOBAL_UNIT_ASSIGNED_CONTEXT((#4995,#4997,#4998))
REPRESENTATION_CONTEXT('','3D')
);
#4995=(
LENGTH_UNIT()
NAMED_UNIT(*)
SI_UNIT(.MILLI.,.METRE.)
);
#4997=(
NAMED_UNIT(*)
PLANE_ANGLE_UNIT()
SI_UNIT($,.RADIAN.)
);
#4998=(
NAMED_UNIT(*)
SI_UNIT($,.STERADIAN.)
SOLID_ANGLE_UNIT()
);
#5005=SHAPE_DEFINITION_REPRESENTATION(#5016,#5037);
#5016=PRODUCT_DEFINITION_SHAPE('',$,#5049);
#5037=SHAPE_REPRESENTATION('',(#3203),#4989);
#5042=PRODUCT_DEFINITION_CONTEXT('part definition',#5077,'design');
#5049=PRODUCT_DEFINITION('Carriage','Carriage',#5060,#5042);
#5060=PRODUCT_DEFINITION_FORMATION('',$,#5085);
#5077=APPLICATION_CONTEXT(
'Core Data for Automotive Mechanical Design Process');
#5078=PRODUCT_CONTEXT('part definition',#5077,'mechanical');
#5085=PRODUCT('Carriage','Carriage',$,(#5078));
#5092=PRESENTATION_STYLE_ASSIGNMENT((#5097));
#5097=SURFACE_STYLE_USAGE(.BOTH.,#5102);
#5102=SURFACE_SIDE_STYLE('',(#5107));
#5107=SURFACE_STYLE_FILL_AREA(#5112);
#5112=FILL_AREA_STYLE('Opaque(211,211,211)',(#5117));
#5117=FILL_AREA_STYLE_COLOUR('Opaque(211,211,211)',#5122);
#5122=COLOUR_RGB('Opaque(211,211,211)', 0.72549020, 0.75294118, 0.79215686);
ENDSEC;
END-ISO-10303-21;
